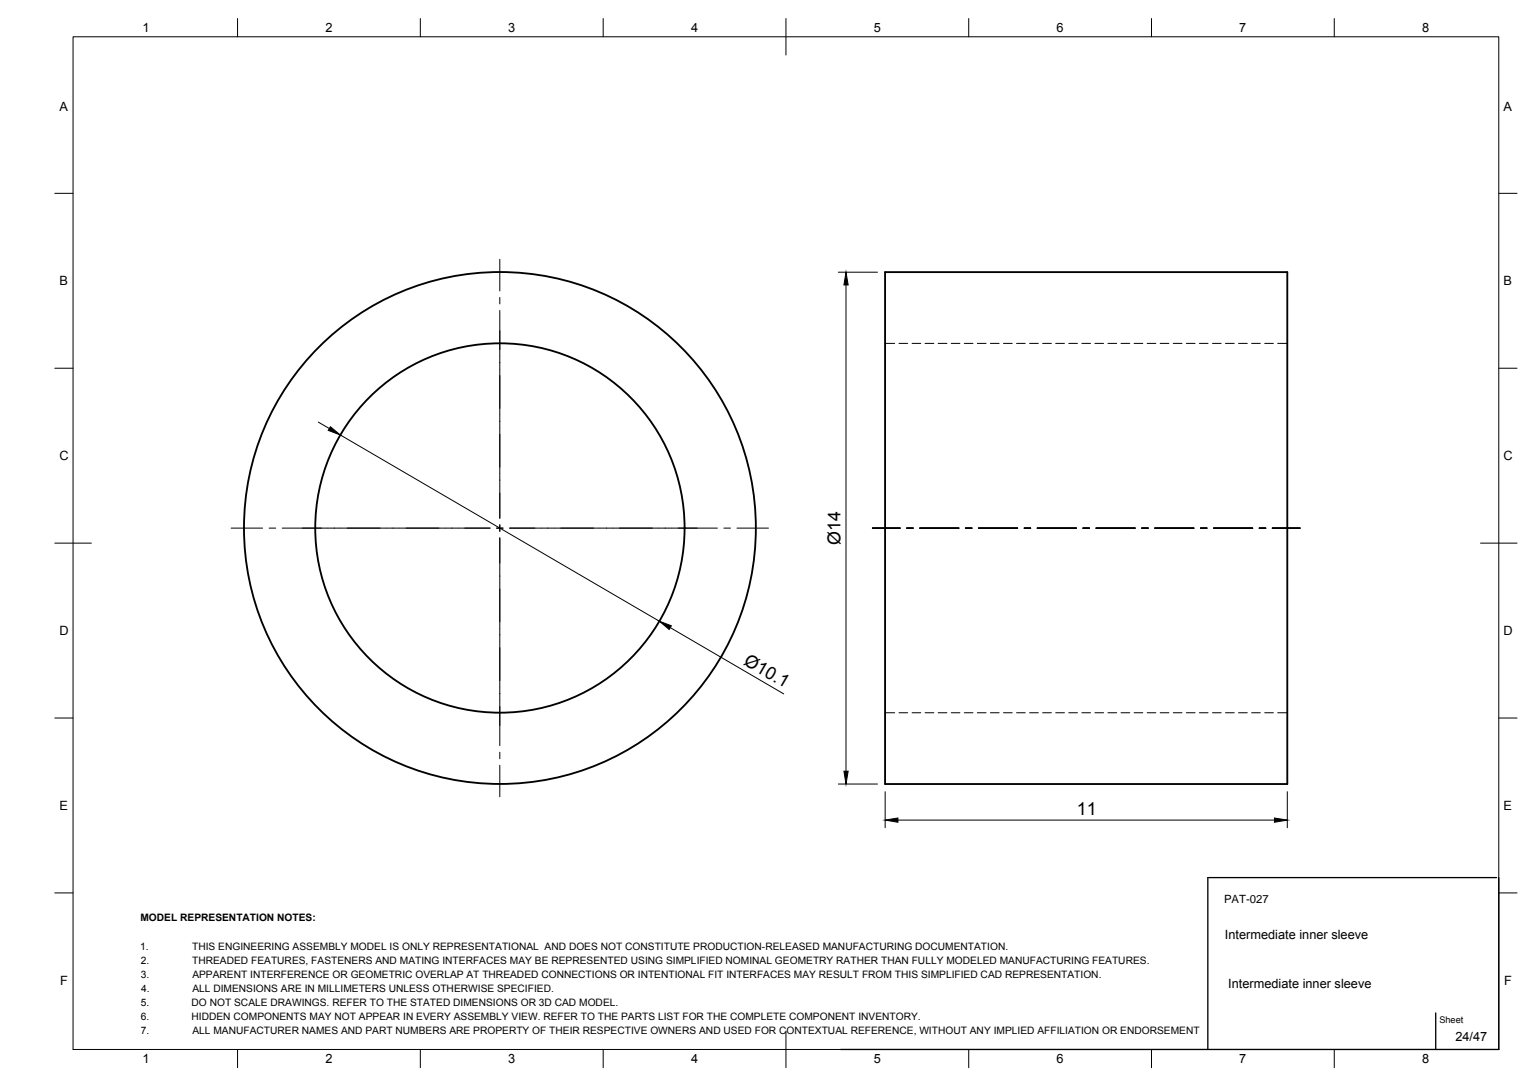
ISO-10303-21;
HEADER;
/* Generated by software containing ST-Developer
 * from STEP Tools, Inc. (www.steptools.com) 
 */

FILE_DESCRIPTION(
/* description */ ('Crank-driven oscillating fan base (mechanism only)'),

/* implementation_level */ '2;1');

FILE_NAME(
/* name */ 'Intermediate inner sleeve.step',
/* time_stamp */ '2026-10-28T03:25:00-07:00',
/* author */ (''),
/* organization */ (''),
/* preprocessor_version */ 'ST-DEVELOPER v20.2',
/* originating_system */ 'Autodesk Translation Framework v15.17.0.0',
/* authorisation */ '');

FILE_SCHEMA (('AUTOMOTIVE_DESIGN { 1 0 10303 214 3 1 1 }'));
ENDSEC;

DATA;
#10=MECHANICAL_DESIGN_GEOMETRIC_PRESENTATION_REPRESENTATION('',(#461),#11916);
#373=SHAPE_REPRESENTATION_RELATIONSHIP('SRR','None',#12099,#413);
#413=ADVANCED_BREP_SHAPE_REPRESENTATION('',(#508),#11890);
#461=STYLED_ITEM('',(#12368),#508);
#508=MANIFOLD_SOLID_BREP('Body1',#6092);
#624=FACE_BOUND('',#1552,.T.);
#625=FACE_BOUND('',#1554,.T.);
#780=PLANE('',#7010);
#781=PLANE('',#7011);
#1080=FACE_OUTER_BOUND('',#1549,.T.);
#1081=FACE_OUTER_BOUND('',#1550,.T.);
#1082=FACE_OUTER_BOUND('',#1551,.T.);
#1083=FACE_OUTER_BOUND('',#1553,.T.);
#1549=EDGE_LOOP('',(#4882,#4883,#4884,#4885));
#1550=EDGE_LOOP('',(#4886,#4887,#4888,#4889));
#1551=EDGE_LOOP('',(#4890));
#1552=EDGE_LOOP('',(#4891));
#1553=EDGE_LOOP('',(#4892));
#1554=EDGE_LOOP('',(#4893));
#1954=LINE('',#10834,#2287);
#1955=LINE('',#10840,#2288);
#2287=VECTOR('',#8461,0.505);
#2288=VECTOR('',#8468,0.7);
#2689=CIRCLE('',#7005,0.505);
#2690=CIRCLE('',#7006,0.505);
#2691=CIRCLE('',#7008,0.7);
#2692=CIRCLE('',#7009,0.7);
#3110=VERTEX_POINT('',#10831);
#3111=VERTEX_POINT('',#10833);
#3112=VERTEX_POINT('',#10837);
#3113=VERTEX_POINT('',#10839);
#3736=EDGE_CURVE('',#3110,#3110,#2689,.T.);
#3737=EDGE_CURVE('',#3110,#3111,#1954,.T.);
#3738=EDGE_CURVE('',#3111,#3111,#2690,.T.);
#3739=EDGE_CURVE('',#3112,#3112,#2691,.T.);
#3740=EDGE_CURVE('',#3112,#3113,#1955,.T.);
#3741=EDGE_CURVE('',#3113,#3113,#2692,.T.);
#4882=ORIENTED_EDGE('',*,*,#3736,.F.);
#4883=ORIENTED_EDGE('',*,*,#3737,.T.);
#4884=ORIENTED_EDGE('',*,*,#3738,.T.);
#4885=ORIENTED_EDGE('',*,*,#3737,.F.);
#4886=ORIENTED_EDGE('',*,*,#3739,.F.);
#4887=ORIENTED_EDGE('',*,*,#3740,.T.);
#4888=ORIENTED_EDGE('',*,*,#3741,.T.);
#4889=ORIENTED_EDGE('',*,*,#3740,.F.);
#4890=ORIENTED_EDGE('',*,*,#3739,.T.);
#4891=ORIENTED_EDGE('',*,*,#3736,.T.);
#4892=ORIENTED_EDGE('',*,*,#3741,.F.);
#4893=ORIENTED_EDGE('',*,*,#3738,.F.);
#5627=CYLINDRICAL_SURFACE('',#7004,0.505);
#5628=CYLINDRICAL_SURFACE('',#7007,0.7);
#5886=ADVANCED_FACE('',(#1080),#5627,.F.);
#5887=ADVANCED_FACE('',(#1081),#5628,.T.);
#5888=ADVANCED_FACE('',(#1082,#624),#780,.T.);
#5889=ADVANCED_FACE('',(#1083,#625),#781,.F.);
#6092=CLOSED_SHELL('',(#5886,#5887,#5888,#5889));
#7003=AXIS2_PLACEMENT_3D('',#10829,#8455,#8456);
#7004=AXIS2_PLACEMENT_3D('',#10830,#8457,#8458);
#7005=AXIS2_PLACEMENT_3D('',#10832,#8459,#8460);
#7006=AXIS2_PLACEMENT_3D('',#10835,#8462,#8463);
#7007=AXIS2_PLACEMENT_3D('',#10836,#8464,#8465);
#7008=AXIS2_PLACEMENT_3D('',#10838,#8466,#8467);
#7009=AXIS2_PLACEMENT_3D('',#10841,#8469,#8470);
#7010=AXIS2_PLACEMENT_3D('',#10842,#8471,#8472);
#7011=AXIS2_PLACEMENT_3D('',#10843,#8473,#8474);
#8455=DIRECTION('axis',(0.,0.,1.));
#8456=DIRECTION('refdir',(1.,0.,0.));
#8457=DIRECTION('center_axis',(0.,0.,1.));
#8458=DIRECTION('ref_axis',(1.,0.,0.));
#8459=DIRECTION('center_axis',(0.,0.,-1.));
#8460=DIRECTION('ref_axis',(1.,0.,0.));
#8461=DIRECTION('',(0.,0.,-1.));
#8462=DIRECTION('center_axis',(0.,0.,-1.));
#8463=DIRECTION('ref_axis',(1.,0.,0.));
#8464=DIRECTION('center_axis',(0.,0.,1.));
#8465=DIRECTION('ref_axis',(1.,0.,0.));
#8466=DIRECTION('center_axis',(0.,0.,1.));
#8467=DIRECTION('ref_axis',(1.,0.,0.));
#8468=DIRECTION('',(0.,0.,-1.));
#8469=DIRECTION('center_axis',(0.,0.,1.));
#8470=DIRECTION('ref_axis',(1.,0.,0.));
#8471=DIRECTION('center_axis',(0.,0.,1.));
#8472=DIRECTION('ref_axis',(1.,0.,0.));
#8473=DIRECTION('center_axis',(0.,0.,1.));
#8474=DIRECTION('ref_axis',(1.,0.,0.));
#10829=CARTESIAN_POINT('',(0.,0.,0.));
#10830=CARTESIAN_POINT('Origin',(0.,0.,2.95));
#10831=CARTESIAN_POINT('',(-0.505,-6.18446633569413E-17,4.05));
#10832=CARTESIAN_POINT('Origin',(0.,0.,4.05));
#10833=CARTESIAN_POINT('',(-0.505,-6.18446633569413E-17,2.95));
#10834=CARTESIAN_POINT('',(-0.505,-6.18446633569413E-17,2.95));
#10835=CARTESIAN_POINT('Origin',(0.,0.,2.95));
#10836=CARTESIAN_POINT('Origin',(0.,0.,2.95));
#10837=CARTESIAN_POINT('',(-0.7,-8.57252759403147E-17,4.05));
#10838=CARTESIAN_POINT('Origin',(0.,0.,4.05));
#10839=CARTESIAN_POINT('',(-0.7,-8.57252759403147E-17,2.95));
#10840=CARTESIAN_POINT('',(-0.7,-8.57252759403147E-17,2.95));
#10841=CARTESIAN_POINT('Origin',(0.,0.,2.95));
#10842=CARTESIAN_POINT('Origin',(0.,0.,4.05));
#10843=CARTESIAN_POINT('Origin',(0.,0.,2.95));
#11843=UNCERTAINTY_MEASURE_WITH_UNIT(LENGTH_MEASURE(0.001),#11917,
'DISTANCE_ACCURACY_VALUE',
'Maximum model space distance between geometric entities at asserted c
onnectivities');
#11869=UNCERTAINTY_MEASURE_WITH_UNIT(LENGTH_MEASURE(0.001),#11917,
'DISTANCE_ACCURACY_VALUE',
'Maximum model space distance between geometric entities at asserted c
onnectivities');
#11890=(
GEOMETRIC_REPRESENTATION_CONTEXT(3)
GLOBAL_UNCERTAINTY_ASSIGNED_CONTEXT((#11843))
GLOBAL_UNIT_ASSIGNED_CONTEXT((#11917,#11919,#11920))
REPRESENTATION_CONTEXT('','3D')
);
#11916=(
GEOMETRIC_REPRESENTATION_CONTEXT(3)
GLOBAL_UNCERTAINTY_ASSIGNED_CONTEXT((#11869))
GLOBAL_UNIT_ASSIGNED_CONTEXT((#11917,#11919,#11920))
REPRESENTATION_CONTEXT('','3D')
);
#11917=(
LENGTH_UNIT()
NAMED_UNIT(*)
SI_UNIT(.CENTI.,.METRE.)
);
#11919=(
NAMED_UNIT(*)
PLANE_ANGLE_UNIT()
SI_UNIT($,.RADIAN.)
);
#11920=(
NAMED_UNIT(*)
SI_UNIT($,.STERADIAN.)
SOLID_ANGLE_UNIT()
);
#11941=SHAPE_DEFINITION_REPRESENTATION(#11992,#12099);
#11992=PRODUCT_DEFINITION_SHAPE('',$,#12146);
#12099=SHAPE_REPRESENTATION('',(#7003),#11890);
#12125=PRODUCT_DEFINITION_CONTEXT('part definition',#12265,'design');
#12146=PRODUCT_DEFINITION('Intermediate inner sleeve',
'Intermediate inner sleeve',#12192,#12125);
#12192=PRODUCT_DEFINITION_FORMATION('',$,#12287);
#12265=APPLICATION_CONTEXT(
'Core Data for Automotive Mechanical Design Process');
#12266=PRODUCT_CONTEXT('part definition',#12265,'mechanical');
#12287=PRODUCT('Intermediate inner sleeve','Intermediate inner sleeve',
'Intermediate inner sleeve',(#12266));
#12362=COLOUR_RGB('Sky Blue',0.24,0.69,0.87);
#12363=FILL_AREA_STYLE_COLOUR('',#12362);
#12364=FILL_AREA_STYLE('',(#12363));
#12365=SURFACE_STYLE_FILL_AREA(#12364);
#12366=SURFACE_SIDE_STYLE('',(#12365));
#12367=SURFACE_STYLE_USAGE(.BOTH.,#12366);
#12368=PRESENTATION_STYLE_ASSIGNMENT((#12367));
ENDSEC;
END-ISO-10303-21;
